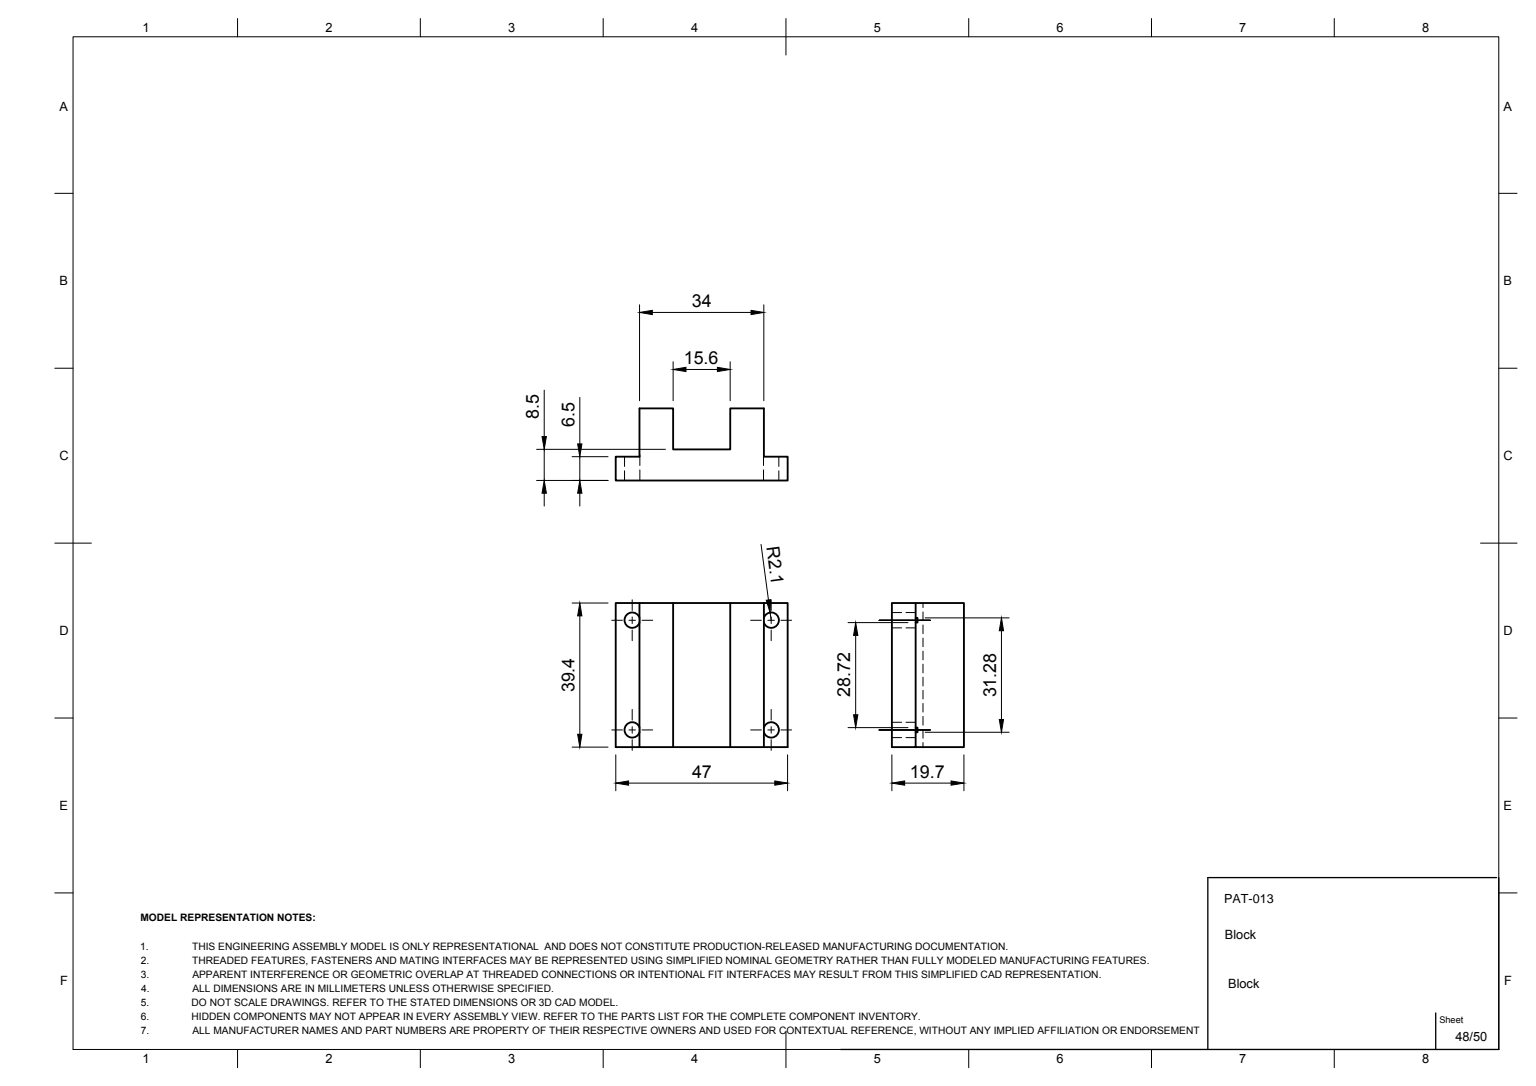
ISO-10303-21;
HEADER;
/* Generated by software containing ST-Developer
 * from STEP Tools, Inc. (www.steptools.com) 
 */

FILE_DESCRIPTION(
/* description */ ('Belt-driven linear axis on 2020 extrusion'),
/* implementation_level */ '2;1');

FILE_NAME(
/* name */ 'Block.step',
/* time_stamp */ '2026-10-28T03:26:09-07:00',
/* author */ (''),
/* organization */ (''),
/* preprocessor_version */ 'ST-DEVELOPER v20.2',
/* originating_system */ 'Autodesk Translation Framework v15.17.0.0',
/* authorisation */ '');

FILE_SCHEMA (('AUTOMOTIVE_DESIGN { 1 0 10303 214 3 1 1 }'));
ENDSEC;

DATA;
#10=MECHANICAL_DESIGN_GEOMETRIC_PRESENTATION_REPRESENTATION('',(#659),#20096);
#557=SHAPE_REPRESENTATION_RELATIONSHIP('SRR','None',#20358,#603);
#603=ADVANCED_BREP_SHAPE_REPRESENTATION('',(#714),#20089);
#659=STYLED_ITEM('',(#20629),#714);
#714=MANIFOLD_SOLID_BREP('Body1',#10973);
#880=FACE_BOUND('',#2573,.T.);
#881=FACE_BOUND('',#2574,.T.);
#882=FACE_BOUND('',#2575,.T.);
#883=FACE_BOUND('',#2576,.T.);
#1177=PLANE('',#12538);
#1178=PLANE('',#12544);
#1179=PLANE('',#12550);
#1180=PLANE('',#12556);
#1181=PLANE('',#12562);
#1182=PLANE('',#12563);
#1183=PLANE('',#12564);
#1184=PLANE('',#12565);
#1185=PLANE('',#12566);
#1186=PLANE('',#12567);
#1187=PLANE('',#12568);
#1188=PLANE('',#12569);
#1189=PLANE('',#12570);
#1190=PLANE('',#12571);
#1191=PLANE('',#12572);
#1192=PLANE('',#12573);
#1193=PLANE('',#12574);
#1194=PLANE('',#12575);
#1775=FACE_OUTER_BOUND('',#2559,.T.);
#1776=FACE_OUTER_BOUND('',#2560,.T.);
#1777=FACE_OUTER_BOUND('',#2561,.T.);
#1778=FACE_OUTER_BOUND('',#2562,.T.);
#1779=FACE_OUTER_BOUND('',#2563,.T.);
#1780=FACE_OUTER_BOUND('',#2564,.T.);
#1781=FACE_OUTER_BOUND('',#2565,.T.);
#1782=FACE_OUTER_BOUND('',#2566,.T.);
#1783=FACE_OUTER_BOUND('',#2567,.T.);
#1784=FACE_OUTER_BOUND('',#2568,.T.);
#1785=FACE_OUTER_BOUND('',#2569,.T.);
#1786=FACE_OUTER_BOUND('',#2570,.T.);
#1787=FACE_OUTER_BOUND('',#2571,.T.);
#1788=FACE_OUTER_BOUND('',#2572,.T.);
#1789=FACE_OUTER_BOUND('',#2577,.T.);
#1790=FACE_OUTER_BOUND('',#2578,.T.);
#1791=FACE_OUTER_BOUND('',#2579,.T.);
#1792=FACE_OUTER_BOUND('',#2580,.T.);
#1793=FACE_OUTER_BOUND('',#2581,.T.);
#1794=FACE_OUTER_BOUND('',#2582,.T.);
#1795=FACE_OUTER_BOUND('',#2583,.T.);
#1796=FACE_OUTER_BOUND('',#2584,.T.);
#2559=EDGE_LOOP('',(#9633,#9634));
#2560=EDGE_LOOP('',(#9635,#9636,#9637,#9638,#9639,#9640,#9641,#9642));
#2561=EDGE_LOOP('',(#9643,#9644));
#2562=EDGE_LOOP('',(#9645,#9646,#9647,#9648,#9649,#9650,#9651,#9652));
#2563=EDGE_LOOP('',(#9653,#9654));
#2564=EDGE_LOOP('',(#9655,#9656,#9657,#9658,#9659,#9660,#9661,#9662));
#2565=EDGE_LOOP('',(#9663,#9664));
#2566=EDGE_LOOP('',(#9665,#9666,#9667,#9668,#9669,#9670,#9671,#9672));
#2567=EDGE_LOOP('',(#9673,#9674,#9675,#9676,#9677,#9678,#9679,#9680,#9681,
#9682,#9683,#9684));
#2568=EDGE_LOOP('',(#9685,#9686,#9687,#9688,#9689,#9690,#9691,#9692,#9693,
#9694,#9695,#9696));
#2569=EDGE_LOOP('',(#9697,#9698,#9699,#9700,#9701,#9702,#9703,#9704,#9705,
#9706,#9707,#9708));
#2570=EDGE_LOOP('',(#9709,#9710,#9711,#9712,#9713,#9714,#9715,#9716,#9717,
#9718));
#2571=EDGE_LOOP('',(#9719,#9720,#9721,#9722));
#2572=EDGE_LOOP('',(#9723,#9724,#9725,#9726));
#2573=EDGE_LOOP('',(#9727));
#2574=EDGE_LOOP('',(#9728));
#2575=EDGE_LOOP('',(#9729));
#2576=EDGE_LOOP('',(#9730));
#2577=EDGE_LOOP('',(#9731,#9732,#9733,#9734));
#2578=EDGE_LOOP('',(#9735,#9736,#9737,#9738,#9739,#9740,#9741,#9742,#9743,
#9744));
#2579=EDGE_LOOP('',(#9745,#9746,#9747,#9748));
#2580=EDGE_LOOP('',(#9749,#9750,#9751,#9752));
#2581=EDGE_LOOP('',(#9753,#9754,#9755,#9756));
#2582=EDGE_LOOP('',(#9757,#9758,#9759,#9760));
#2583=EDGE_LOOP('',(#9761,#9762,#9763,#9764));
#2584=EDGE_LOOP('',(#9765,#9766,#9767,#9768,#9769,#9770,#9771,#9772,#9773,
#9774,#9775,#9776));
#3344=LINE('',#19423,#4201);
#3345=LINE('',#19427,#4202);
#3346=LINE('',#19431,#4203);
#3347=LINE('',#19435,#4204);
#3348=LINE('',#19439,#4205);
#3349=LINE('',#19443,#4206);
#3350=LINE('',#19447,#4207);
#3351=LINE('',#19451,#4208);
#3352=LINE('',#19455,#4209);
#3353=LINE('',#19459,#4210);
#3354=LINE('',#19463,#4211);
#3355=LINE('',#19467,#4212);
#3356=LINE('',#19471,#4213);
#3357=LINE('',#19475,#4214);
#3358=LINE('',#19479,#4215);
#3359=LINE('',#19483,#4216);
#3360=LINE('',#19485,#4217);
#3361=LINE('',#19487,#4218);
#3362=LINE('',#19489,#4219);
#3363=LINE('',#19491,#4220);
#3364=LINE('',#19493,#4221);
#3365=LINE('',#19494,#4222);
#3366=LINE('',#19496,#4223);
#3367=LINE('',#19498,#4224);
#3368=LINE('',#19500,#4225);
#3369=LINE('',#19502,#4226);
#3370=LINE('',#19504,#4227);
#3371=LINE('',#19505,#4228);
#3372=LINE('',#19508,#4229);
#3373=LINE('',#19510,#4230);
#3374=LINE('',#19512,#4231);
#3375=LINE('',#19514,#4232);
#3376=LINE('',#19515,#4233);
#3377=LINE('',#19517,#4234);
#3378=LINE('',#19519,#4235);
#3379=LINE('',#19521,#4236);
#3380=LINE('',#19523,#4237);
#3381=LINE('',#19524,#4238);
#3382=LINE('',#19527,#4239);
#3383=LINE('',#19528,#4240);
#3384=LINE('',#19531,#4241);
#3385=LINE('',#19532,#4242);
#3386=LINE('',#19535,#4243);
#3387=LINE('',#19536,#4244);
#3388=LINE('',#19539,#4245);
#3389=LINE('',#19540,#4246);
#3390=LINE('',#19542,#4247);
#3391=LINE('',#19545,#4248);
#3392=LINE('',#19546,#4249);
#3393=LINE('',#19549,#4250);
#3394=LINE('',#19550,#4251);
#3395=LINE('',#19553,#4252);
#3396=LINE('',#19554,#4253);
#3397=LINE('',#19557,#4254);
#3398=LINE('',#19558,#4255);
#3399=LINE('',#19560,#4256);
#4201=VECTOR('',#15562,1.);
#4202=VECTOR('',#15567,1.);
#4203=VECTOR('',#15570,0.21);
#4204=VECTOR('',#15575,1.);
#4205=VECTOR('',#15578,1.);
#4206=VECTOR('',#15583,1.);
#4207=VECTOR('',#15586,0.21);
#4208=VECTOR('',#15591,1.);
#4209=VECTOR('',#15594,1.);
#4210=VECTOR('',#15599,1.);
#4211=VECTOR('',#15602,0.21);
#4212=VECTOR('',#15607,1.);
#4213=VECTOR('',#15610,1.);
#4214=VECTOR('',#15615,1.);
#4215=VECTOR('',#15618,0.21);
#4216=VECTOR('',#15623,1.);
#4217=VECTOR('',#15626,1.);
#4218=VECTOR('',#15627,1.);
#4219=VECTOR('',#15628,1.);
#4220=VECTOR('',#15629,1.);
#4221=VECTOR('',#15630,1.);
#4222=VECTOR('',#15631,1.);
#4223=VECTOR('',#15634,1.);
#4224=VECTOR('',#15635,1.);
#4225=VECTOR('',#15636,1.);
#4226=VECTOR('',#15637,1.);
#4227=VECTOR('',#15638,1.);
#4228=VECTOR('',#15639,1.);
#4229=VECTOR('',#15642,1.);
#4230=VECTOR('',#15643,1.);
#4231=VECTOR('',#15644,1.);
#4232=VECTOR('',#15645,1.);
#4233=VECTOR('',#15646,1.);
#4234=VECTOR('',#15647,1.);
#4235=VECTOR('',#15648,1.);
#4236=VECTOR('',#15649,1.);
#4237=VECTOR('',#15650,1.);
#4238=VECTOR('',#15651,1.);
#4239=VECTOR('',#15654,1.);
#4240=VECTOR('',#15655,1.);
#4241=VECTOR('',#15658,1.);
#4242=VECTOR('',#15659,1.);
#4243=VECTOR('',#15662,1.);
#4244=VECTOR('',#15663,1.);
#4245=VECTOR('',#15666,1.);
#4246=VECTOR('',#15667,1.);
#4247=VECTOR('',#15670,1.);
#4248=VECTOR('',#15673,1.);
#4249=VECTOR('',#15674,1.);
#4250=VECTOR('',#15677,1.);
#4251=VECTOR('',#15678,1.);
#4252=VECTOR('',#15681,1.);
#4253=VECTOR('',#15682,1.);
#4254=VECTOR('',#15685,1.);
#4255=VECTOR('',#15686,1.);
#4256=VECTOR('',#15689,1.);
#4848=CIRCLE('',#12539,0.21);
#4849=CIRCLE('',#12541,0.21);
#4850=CIRCLE('',#12542,0.21);
#4851=CIRCLE('',#12543,0.21);
#4852=CIRCLE('',#12545,0.21);
#4853=CIRCLE('',#12547,0.21);
#4854=CIRCLE('',#12548,0.21);
#4855=CIRCLE('',#12549,0.21);
#4856=CIRCLE('',#12551,0.21);
#4857=CIRCLE('',#12553,0.21);
#4858=CIRCLE('',#12554,0.21);
#4859=CIRCLE('',#12555,0.21);
#4860=CIRCLE('',#12557,0.21);
#4861=CIRCLE('',#12559,0.21);
#4862=CIRCLE('',#12560,0.21);
#4863=CIRCLE('',#12561,0.21);
#5697=VERTEX_POINT('',#19421);
#5698=VERTEX_POINT('',#19422);
#5699=VERTEX_POINT('',#19426);
#5700=VERTEX_POINT('',#19428);
#5701=VERTEX_POINT('',#19430);
#5702=VERTEX_POINT('',#19433);
#5703=VERTEX_POINT('',#19437);
#5704=VERTEX_POINT('',#19438);
#5705=VERTEX_POINT('',#19442);
#5706=VERTEX_POINT('',#19444);
#5707=VERTEX_POINT('',#19446);
#5708=VERTEX_POINT('',#19449);
#5709=VERTEX_POINT('',#19453);
#5710=VERTEX_POINT('',#19454);
#5711=VERTEX_POINT('',#19458);
#5712=VERTEX_POINT('',#19460);
#5713=VERTEX_POINT('',#19462);
#5714=VERTEX_POINT('',#19465);
#5715=VERTEX_POINT('',#19469);
#5716=VERTEX_POINT('',#19470);
#5717=VERTEX_POINT('',#19474);
#5718=VERTEX_POINT('',#19476);
#5719=VERTEX_POINT('',#19478);
#5720=VERTEX_POINT('',#19481);
#5721=VERTEX_POINT('',#19486);
#5722=VERTEX_POINT('',#19488);
#5723=VERTEX_POINT('',#19490);
#5724=VERTEX_POINT('',#19492);
#5725=VERTEX_POINT('',#19497);
#5726=VERTEX_POINT('',#19499);
#5727=VERTEX_POINT('',#19501);
#5728=VERTEX_POINT('',#19503);
#5729=VERTEX_POINT('',#19507);
#5730=VERTEX_POINT('',#19509);
#5731=VERTEX_POINT('',#19511);
#5732=VERTEX_POINT('',#19513);
#5733=VERTEX_POINT('',#19516);
#5734=VERTEX_POINT('',#19518);
#5735=VERTEX_POINT('',#19520);
#5736=VERTEX_POINT('',#19522);
#5737=VERTEX_POINT('',#19526);
#5738=VERTEX_POINT('',#19530);
#5739=VERTEX_POINT('',#19534);
#5740=VERTEX_POINT('',#19538);
#5741=VERTEX_POINT('',#19544);
#5742=VERTEX_POINT('',#19548);
#5743=VERTEX_POINT('',#19552);
#5744=VERTEX_POINT('',#19556);
#7031=EDGE_CURVE('',#5697,#5698,#3344,.T.);
#7032=EDGE_CURVE('',#5697,#5698,#4848,.T.);
#7033=EDGE_CURVE('',#5699,#5697,#3345,.T.);
#7034=EDGE_CURVE('',#5700,#5699,#4849,.T.);
#7035=EDGE_CURVE('',#5700,#5701,#3346,.T.);
#7036=EDGE_CURVE('',#5701,#5701,#4850,.T.);
#7037=EDGE_CURVE('',#5702,#5700,#4851,.T.);
#7038=EDGE_CURVE('',#5698,#5702,#3347,.T.);
#7039=EDGE_CURVE('',#5703,#5704,#3348,.T.);
#7040=EDGE_CURVE('',#5703,#5704,#4852,.T.);
#7041=EDGE_CURVE('',#5705,#5703,#3349,.T.);
#7042=EDGE_CURVE('',#5706,#5705,#4853,.T.);
#7043=EDGE_CURVE('',#5706,#5707,#3350,.T.);
#7044=EDGE_CURVE('',#5707,#5707,#4854,.T.);
#7045=EDGE_CURVE('',#5708,#5706,#4855,.T.);
#7046=EDGE_CURVE('',#5704,#5708,#3351,.T.);
#7047=EDGE_CURVE('',#5709,#5710,#3352,.T.);
#7048=EDGE_CURVE('',#5709,#5710,#4856,.T.);
#7049=EDGE_CURVE('',#5711,#5709,#3353,.T.);
#7050=EDGE_CURVE('',#5712,#5711,#4857,.T.);
#7051=EDGE_CURVE('',#5712,#5713,#3354,.T.);
#7052=EDGE_CURVE('',#5713,#5713,#4858,.T.);
#7053=EDGE_CURVE('',#5714,#5712,#4859,.T.);
#7054=EDGE_CURVE('',#5710,#5714,#3355,.T.);
#7055=EDGE_CURVE('',#5715,#5716,#3356,.T.);
#7056=EDGE_CURVE('',#5715,#5716,#4860,.T.);
#7057=EDGE_CURVE('',#5717,#5715,#3357,.T.);
#7058=EDGE_CURVE('',#5718,#5717,#4861,.T.);
#7059=EDGE_CURVE('',#5718,#5719,#3358,.T.);
#7060=EDGE_CURVE('',#5719,#5719,#4862,.T.);
#7061=EDGE_CURVE('',#5720,#5718,#4863,.T.);
#7062=EDGE_CURVE('',#5716,#5720,#3359,.T.);
#7063=EDGE_CURVE('',#5702,#5711,#3360,.T.);
#7064=EDGE_CURVE('',#5714,#5721,#3361,.T.);
#7065=EDGE_CURVE('',#5722,#5721,#3362,.T.);
#7066=EDGE_CURVE('',#5722,#5723,#3363,.T.);
#7067=EDGE_CURVE('',#5724,#5723,#3364,.T.);
#7068=EDGE_CURVE('',#5724,#5699,#3365,.T.);
#7069=EDGE_CURVE('',#5708,#5717,#3366,.T.);
#7070=EDGE_CURVE('',#5720,#5725,#3367,.T.);
#7071=EDGE_CURVE('',#5726,#5725,#3368,.T.);
#7072=EDGE_CURVE('',#5727,#5726,#3369,.T.);
#7073=EDGE_CURVE('',#5728,#5727,#3370,.T.);
#7074=EDGE_CURVE('',#5728,#5705,#3371,.T.);
#7075=EDGE_CURVE('',#5721,#5729,#3372,.T.);
#7076=EDGE_CURVE('',#5729,#5730,#3373,.T.);
#7077=EDGE_CURVE('',#5730,#5731,#3374,.T.);
#7078=EDGE_CURVE('',#5731,#5732,#3375,.T.);
#7079=EDGE_CURVE('',#5732,#5728,#3376,.T.);
#7080=EDGE_CURVE('',#5727,#5733,#3377,.T.);
#7081=EDGE_CURVE('',#5733,#5734,#3378,.T.);
#7082=EDGE_CURVE('',#5734,#5735,#3379,.T.);
#7083=EDGE_CURVE('',#5735,#5736,#3380,.T.);
#7084=EDGE_CURVE('',#5736,#5722,#3381,.T.);
#7085=EDGE_CURVE('',#5737,#5724,#3382,.T.);
#7086=EDGE_CURVE('',#5729,#5737,#3383,.T.);
#7087=EDGE_CURVE('',#5738,#5737,#3384,.T.);
#7088=EDGE_CURVE('',#5730,#5738,#3385,.T.);
#7089=EDGE_CURVE('',#5739,#5738,#3386,.T.);
#7090=EDGE_CURVE('',#5731,#5739,#3387,.T.);
#7091=EDGE_CURVE('',#5740,#5739,#3388,.T.);
#7092=EDGE_CURVE('',#5732,#5740,#3389,.T.);
#7093=EDGE_CURVE('',#5725,#5740,#3390,.T.);
#7094=EDGE_CURVE('',#5741,#5726,#3391,.T.);
#7095=EDGE_CURVE('',#5733,#5741,#3392,.T.);
#7096=EDGE_CURVE('',#5742,#5741,#3393,.T.);
#7097=EDGE_CURVE('',#5734,#5742,#3394,.T.);
#7098=EDGE_CURVE('',#5743,#5742,#3395,.T.);
#7099=EDGE_CURVE('',#5735,#5743,#3396,.T.);
#7100=EDGE_CURVE('',#5744,#5743,#3397,.T.);
#7101=EDGE_CURVE('',#5736,#5744,#3398,.T.);
#7102=EDGE_CURVE('',#5723,#5744,#3399,.T.);
#9633=ORIENTED_EDGE('',*,*,#7031,.F.);
#9634=ORIENTED_EDGE('',*,*,#7032,.T.);
#9635=ORIENTED_EDGE('',*,*,#7033,.F.);
#9636=ORIENTED_EDGE('',*,*,#7034,.F.);
#9637=ORIENTED_EDGE('',*,*,#7035,.T.);
#9638=ORIENTED_EDGE('',*,*,#7036,.F.);
#9639=ORIENTED_EDGE('',*,*,#7035,.F.);
#9640=ORIENTED_EDGE('',*,*,#7037,.F.);
#9641=ORIENTED_EDGE('',*,*,#7038,.F.);
#9642=ORIENTED_EDGE('',*,*,#7032,.F.);
#9643=ORIENTED_EDGE('',*,*,#7039,.F.);
#9644=ORIENTED_EDGE('',*,*,#7040,.T.);
#9645=ORIENTED_EDGE('',*,*,#7041,.F.);
#9646=ORIENTED_EDGE('',*,*,#7042,.F.);
#9647=ORIENTED_EDGE('',*,*,#7043,.T.);
#9648=ORIENTED_EDGE('',*,*,#7044,.F.);
#9649=ORIENTED_EDGE('',*,*,#7043,.F.);
#9650=ORIENTED_EDGE('',*,*,#7045,.F.);
#9651=ORIENTED_EDGE('',*,*,#7046,.F.);
#9652=ORIENTED_EDGE('',*,*,#7040,.F.);
#9653=ORIENTED_EDGE('',*,*,#7047,.F.);
#9654=ORIENTED_EDGE('',*,*,#7048,.T.);
#9655=ORIENTED_EDGE('',*,*,#7049,.F.);
#9656=ORIENTED_EDGE('',*,*,#7050,.F.);
#9657=ORIENTED_EDGE('',*,*,#7051,.T.);
#9658=ORIENTED_EDGE('',*,*,#7052,.F.);
#9659=ORIENTED_EDGE('',*,*,#7051,.F.);
#9660=ORIENTED_EDGE('',*,*,#7053,.F.);
#9661=ORIENTED_EDGE('',*,*,#7054,.F.);
#9662=ORIENTED_EDGE('',*,*,#7048,.F.);
#9663=ORIENTED_EDGE('',*,*,#7055,.F.);
#9664=ORIENTED_EDGE('',*,*,#7056,.T.);
#9665=ORIENTED_EDGE('',*,*,#7057,.F.);
#9666=ORIENTED_EDGE('',*,*,#7058,.F.);
#9667=ORIENTED_EDGE('',*,*,#7059,.T.);
#9668=ORIENTED_EDGE('',*,*,#7060,.F.);
#9669=ORIENTED_EDGE('',*,*,#7059,.F.);
#9670=ORIENTED_EDGE('',*,*,#7061,.F.);
#9671=ORIENTED_EDGE('',*,*,#7062,.F.);
#9672=ORIENTED_EDGE('',*,*,#7056,.F.);
#9673=ORIENTED_EDGE('',*,*,#7033,.T.);
#9674=ORIENTED_EDGE('',*,*,#7031,.T.);
#9675=ORIENTED_EDGE('',*,*,#7038,.T.);
#9676=ORIENTED_EDGE('',*,*,#7063,.T.);
#9677=ORIENTED_EDGE('',*,*,#7049,.T.);
#9678=ORIENTED_EDGE('',*,*,#7047,.T.);
#9679=ORIENTED_EDGE('',*,*,#7054,.T.);
#9680=ORIENTED_EDGE('',*,*,#7064,.T.);
#9681=ORIENTED_EDGE('',*,*,#7065,.F.);
#9682=ORIENTED_EDGE('',*,*,#7066,.T.);
#9683=ORIENTED_EDGE('',*,*,#7067,.F.);
#9684=ORIENTED_EDGE('',*,*,#7068,.T.);
#9685=ORIENTED_EDGE('',*,*,#7041,.T.);
#9686=ORIENTED_EDGE('',*,*,#7039,.T.);
#9687=ORIENTED_EDGE('',*,*,#7046,.T.);
#9688=ORIENTED_EDGE('',*,*,#7069,.T.);
#9689=ORIENTED_EDGE('',*,*,#7057,.T.);
#9690=ORIENTED_EDGE('',*,*,#7055,.T.);
#9691=ORIENTED_EDGE('',*,*,#7062,.T.);
#9692=ORIENTED_EDGE('',*,*,#7070,.T.);
#9693=ORIENTED_EDGE('',*,*,#7071,.F.);
#9694=ORIENTED_EDGE('',*,*,#7072,.F.);
#9695=ORIENTED_EDGE('',*,*,#7073,.F.);
#9696=ORIENTED_EDGE('',*,*,#7074,.T.);
#9697=ORIENTED_EDGE('',*,*,#7065,.T.);
#9698=ORIENTED_EDGE('',*,*,#7075,.T.);
#9699=ORIENTED_EDGE('',*,*,#7076,.T.);
#9700=ORIENTED_EDGE('',*,*,#7077,.T.);
#9701=ORIENTED_EDGE('',*,*,#7078,.T.);
#9702=ORIENTED_EDGE('',*,*,#7079,.T.);
#9703=ORIENTED_EDGE('',*,*,#7073,.T.);
#9704=ORIENTED_EDGE('',*,*,#7080,.T.);
#9705=ORIENTED_EDGE('',*,*,#7081,.T.);
#9706=ORIENTED_EDGE('',*,*,#7082,.T.);
#9707=ORIENTED_EDGE('',*,*,#7083,.T.);
#9708=ORIENTED_EDGE('',*,*,#7084,.T.);
#9709=ORIENTED_EDGE('',*,*,#7037,.T.);
#9710=ORIENTED_EDGE('',*,*,#7034,.T.);
#9711=ORIENTED_EDGE('',*,*,#7068,.F.);
#9712=ORIENTED_EDGE('',*,*,#7085,.F.);
#9713=ORIENTED_EDGE('',*,*,#7086,.F.);
#9714=ORIENTED_EDGE('',*,*,#7075,.F.);
#9715=ORIENTED_EDGE('',*,*,#7064,.F.);
#9716=ORIENTED_EDGE('',*,*,#7053,.T.);
#9717=ORIENTED_EDGE('',*,*,#7050,.T.);
#9718=ORIENTED_EDGE('',*,*,#7063,.F.);
#9719=ORIENTED_EDGE('',*,*,#7086,.T.);
#9720=ORIENTED_EDGE('',*,*,#7087,.F.);
#9721=ORIENTED_EDGE('',*,*,#7088,.F.);
#9722=ORIENTED_EDGE('',*,*,#7076,.F.);
#9723=ORIENTED_EDGE('',*,*,#7088,.T.);
#9724=ORIENTED_EDGE('',*,*,#7089,.F.);
#9725=ORIENTED_EDGE('',*,*,#7090,.F.);
#9726=ORIENTED_EDGE('',*,*,#7077,.F.);
#9727=ORIENTED_EDGE('',*,*,#7036,.T.);
#9728=ORIENTED_EDGE('',*,*,#7044,.T.);
#9729=ORIENTED_EDGE('',*,*,#7052,.T.);
#9730=ORIENTED_EDGE('',*,*,#7060,.T.);
#9731=ORIENTED_EDGE('',*,*,#7090,.T.);
#9732=ORIENTED_EDGE('',*,*,#7091,.F.);
#9733=ORIENTED_EDGE('',*,*,#7092,.F.);
#9734=ORIENTED_EDGE('',*,*,#7078,.F.);
#9735=ORIENTED_EDGE('',*,*,#7045,.T.);
#9736=ORIENTED_EDGE('',*,*,#7042,.T.);
#9737=ORIENTED_EDGE('',*,*,#7074,.F.);
#9738=ORIENTED_EDGE('',*,*,#7079,.F.);
#9739=ORIENTED_EDGE('',*,*,#7092,.T.);
#9740=ORIENTED_EDGE('',*,*,#7093,.F.);
#9741=ORIENTED_EDGE('',*,*,#7070,.F.);
#9742=ORIENTED_EDGE('',*,*,#7061,.T.);
#9743=ORIENTED_EDGE('',*,*,#7058,.T.);
#9744=ORIENTED_EDGE('',*,*,#7069,.F.);
#9745=ORIENTED_EDGE('',*,*,#7072,.T.);
#9746=ORIENTED_EDGE('',*,*,#7094,.F.);
#9747=ORIENTED_EDGE('',*,*,#7095,.F.);
#9748=ORIENTED_EDGE('',*,*,#7080,.F.);
#9749=ORIENTED_EDGE('',*,*,#7095,.T.);
#9750=ORIENTED_EDGE('',*,*,#7096,.F.);
#9751=ORIENTED_EDGE('',*,*,#7097,.F.);
#9752=ORIENTED_EDGE('',*,*,#7081,.F.);
#9753=ORIENTED_EDGE('',*,*,#7097,.T.);
#9754=ORIENTED_EDGE('',*,*,#7098,.F.);
#9755=ORIENTED_EDGE('',*,*,#7099,.F.);
#9756=ORIENTED_EDGE('',*,*,#7082,.F.);
#9757=ORIENTED_EDGE('',*,*,#7099,.T.);
#9758=ORIENTED_EDGE('',*,*,#7100,.F.);
#9759=ORIENTED_EDGE('',*,*,#7101,.F.);
#9760=ORIENTED_EDGE('',*,*,#7083,.F.);
#9761=ORIENTED_EDGE('',*,*,#7101,.T.);
#9762=ORIENTED_EDGE('',*,*,#7102,.F.);
#9763=ORIENTED_EDGE('',*,*,#7066,.F.);
#9764=ORIENTED_EDGE('',*,*,#7084,.F.);
#9765=ORIENTED_EDGE('',*,*,#7067,.T.);
#9766=ORIENTED_EDGE('',*,*,#7102,.T.);
#9767=ORIENTED_EDGE('',*,*,#7100,.T.);
#9768=ORIENTED_EDGE('',*,*,#7098,.T.);
#9769=ORIENTED_EDGE('',*,*,#7096,.T.);
#9770=ORIENTED_EDGE('',*,*,#7094,.T.);
#9771=ORIENTED_EDGE('',*,*,#7071,.T.);
#9772=ORIENTED_EDGE('',*,*,#7093,.T.);
#9773=ORIENTED_EDGE('',*,*,#7091,.T.);
#9774=ORIENTED_EDGE('',*,*,#7089,.T.);
#9775=ORIENTED_EDGE('',*,*,#7087,.T.);
#9776=ORIENTED_EDGE('',*,*,#7085,.T.);
#10289=CYLINDRICAL_SURFACE('',#12540,0.21);
#10290=CYLINDRICAL_SURFACE('',#12546,0.21);
#10291=CYLINDRICAL_SURFACE('',#12552,0.21);
#10292=CYLINDRICAL_SURFACE('',#12558,0.21);
#10826=ADVANCED_FACE('',(#1775),#1177,.T.);
#10827=ADVANCED_FACE('',(#1776),#10289,.F.);
#10828=ADVANCED_FACE('',(#1777),#1178,.T.);
#10829=ADVANCED_FACE('',(#1778),#10290,.F.);
#10830=ADVANCED_FACE('',(#1779),#1179,.T.);
#10831=ADVANCED_FACE('',(#1780),#10291,.F.);
#10832=ADVANCED_FACE('',(#1781),#1180,.T.);
#10833=ADVANCED_FACE('',(#1782),#10292,.F.);
#10834=ADVANCED_FACE('',(#1783),#1181,.T.);
#10835=ADVANCED_FACE('',(#1784),#1182,.T.);
#10836=ADVANCED_FACE('',(#1785),#1183,.T.);
#10837=ADVANCED_FACE('',(#1786),#1184,.T.);
#10838=ADVANCED_FACE('',(#1787),#1185,.T.);
#10839=ADVANCED_FACE('',(#1788,#880,#881,#882,#883),#1186,.T.);
#10840=ADVANCED_FACE('',(#1789),#1187,.T.);
#10841=ADVANCED_FACE('',(#1790),#1188,.T.);
#10842=ADVANCED_FACE('',(#1791),#1189,.T.);
#10843=ADVANCED_FACE('',(#1792),#1190,.T.);
#10844=ADVANCED_FACE('',(#1793),#1191,.T.);
#10845=ADVANCED_FACE('',(#1794),#1192,.T.);
#10846=ADVANCED_FACE('',(#1795),#1193,.T.);
#10847=ADVANCED_FACE('',(#1796),#1194,.T.);
#10973=CLOSED_SHELL('',(#10826,#10827,#10828,#10829,#10830,#10831,#10832,
#10833,#10834,#10835,#10836,#10837,#10838,#10839,#10840,#10841,#10842,#10843,
#10844,#10845,#10846,#10847));
#12537=AXIS2_PLACEMENT_3D('',#19419,#15558,#15559);
#12538=AXIS2_PLACEMENT_3D('',#19420,#15560,#15561);
#12539=AXIS2_PLACEMENT_3D('',#19424,#15563,#15564);
#12540=AXIS2_PLACEMENT_3D('',#19425,#15565,#15566);
#12541=AXIS2_PLACEMENT_3D('',#19429,#15568,#15569);
#12542=AXIS2_PLACEMENT_3D('',#19432,#15571,#15572);
#12543=AXIS2_PLACEMENT_3D('',#19434,#15573,#15574);
#12544=AXIS2_PLACEMENT_3D('',#19436,#15576,#15577);
#12545=AXIS2_PLACEMENT_3D('',#19440,#15579,#15580);
#12546=AXIS2_PLACEMENT_3D('',#19441,#15581,#15582);
#12547=AXIS2_PLACEMENT_3D('',#19445,#15584,#15585);
#12548=AXIS2_PLACEMENT_3D('',#19448,#15587,#15588);
#12549=AXIS2_PLACEMENT_3D('',#19450,#15589,#15590);
#12550=AXIS2_PLACEMENT_3D('',#19452,#15592,#15593);
#12551=AXIS2_PLACEMENT_3D('',#19456,#15595,#15596);
#12552=AXIS2_PLACEMENT_3D('',#19457,#15597,#15598);
#12553=AXIS2_PLACEMENT_3D('',#19461,#15600,#15601);
#12554=AXIS2_PLACEMENT_3D('',#19464,#15603,#15604);
#12555=AXIS2_PLACEMENT_3D('',#19466,#15605,#15606);
#12556=AXIS2_PLACEMENT_3D('',#19468,#15608,#15609);
#12557=AXIS2_PLACEMENT_3D('',#19472,#15611,#15612);
#12558=AXIS2_PLACEMENT_3D('',#19473,#15613,#15614);
#12559=AXIS2_PLACEMENT_3D('',#19477,#15616,#15617);
#12560=AXIS2_PLACEMENT_3D('',#19480,#15619,#15620);
#12561=AXIS2_PLACEMENT_3D('',#19482,#15621,#15622);
#12562=AXIS2_PLACEMENT_3D('',#19484,#15624,#15625);
#12563=AXIS2_PLACEMENT_3D('',#19495,#15632,#15633);
#12564=AXIS2_PLACEMENT_3D('',#19506,#15640,#15641);
#12565=AXIS2_PLACEMENT_3D('',#19525,#15652,#15653);
#12566=AXIS2_PLACEMENT_3D('',#19529,#15656,#15657);
#12567=AXIS2_PLACEMENT_3D('',#19533,#15660,#15661);
#12568=AXIS2_PLACEMENT_3D('',#19537,#15664,#15665);
#12569=AXIS2_PLACEMENT_3D('',#19541,#15668,#15669);
#12570=AXIS2_PLACEMENT_3D('',#19543,#15671,#15672);
#12571=AXIS2_PLACEMENT_3D('',#19547,#15675,#15676);
#12572=AXIS2_PLACEMENT_3D('',#19551,#15679,#15680);
#12573=AXIS2_PLACEMENT_3D('',#19555,#15683,#15684);
#12574=AXIS2_PLACEMENT_3D('',#19559,#15687,#15688);
#12575=AXIS2_PLACEMENT_3D('',#19561,#15690,#15691);
#15558=DIRECTION('axis',(0.,0.,1.));
#15559=DIRECTION('refdir',(1.,0.,0.));
#15560=DIRECTION('center_axis',(0.,0.,1.));
#15561=DIRECTION('ref_axis',(1.,0.,0.));
#15562=DIRECTION('',(-1.,0.,0.));
#15563=DIRECTION('center_axis',(0.,0.,1.));
#15564=DIRECTION('ref_axis',(1.,0.,0.));
#15565=DIRECTION('center_axis',(0.,0.,1.));
#15566=DIRECTION('ref_axis',(1.,0.,0.));
#15567=DIRECTION('',(0.,0.,-1.));
#15568=DIRECTION('center_axis',(0.,0.,1.));
#15569=DIRECTION('ref_axis',(1.,0.,0.));
#15570=DIRECTION('',(0.,0.,1.));
#15571=DIRECTION('center_axis',(0.,0.,-1.));
#15572=DIRECTION('ref_axis',(1.,0.,0.));
#15573=DIRECTION('center_axis',(0.,0.,1.));
#15574=DIRECTION('ref_axis',(1.,0.,0.));
#15575=DIRECTION('',(0.,0.,1.));
#15576=DIRECTION('center_axis',(0.,0.,1.));
#15577=DIRECTION('ref_axis',(1.,0.,0.));
#15578=DIRECTION('',(1.,0.,0.));
#15579=DIRECTION('center_axis',(0.,0.,1.));
#15580=DIRECTION('ref_axis',(1.,0.,0.));
#15581=DIRECTION('center_axis',(0.,0.,1.));
#15582=DIRECTION('ref_axis',(1.,0.,0.));
#15583=DIRECTION('',(0.,0.,-1.));
#15584=DIRECTION('center_axis',(0.,0.,1.));
#15585=DIRECTION('ref_axis',(1.,0.,0.));
#15586=DIRECTION('',(0.,0.,1.));
#15587=DIRECTION('center_axis',(0.,0.,-1.));
#15588=DIRECTION('ref_axis',(1.,0.,0.));
#15589=DIRECTION('center_axis',(0.,0.,1.));
#15590=DIRECTION('ref_axis',(1.,0.,0.));
#15591=DIRECTION('',(0.,0.,1.));
#15592=DIRECTION('center_axis',(0.,0.,1.));
#15593=DIRECTION('ref_axis',(1.,0.,0.));
#15594=DIRECTION('',(-1.,0.,0.));
#15595=DIRECTION('center_axis',(0.,0.,1.));
#15596=DIRECTION('ref_axis',(1.,0.,0.));
#15597=DIRECTION('center_axis',(0.,0.,1.));
#15598=DIRECTION('ref_axis',(1.,0.,0.));
#15599=DIRECTION('',(0.,0.,-1.));
#15600=DIRECTION('center_axis',(0.,0.,1.));
#15601=DIRECTION('ref_axis',(1.,0.,0.));
#15602=DIRECTION('',(0.,0.,1.));
#15603=DIRECTION('center_axis',(0.,0.,-1.));
#15604=DIRECTION('ref_axis',(1.,0.,0.));
#15605=DIRECTION('center_axis',(0.,0.,1.));
#15606=DIRECTION('ref_axis',(1.,0.,0.));
#15607=DIRECTION('',(0.,0.,1.));
#15608=DIRECTION('center_axis',(0.,0.,1.));
#15609=DIRECTION('ref_axis',(1.,0.,0.));
#15610=DIRECTION('',(1.,0.,0.));
#15611=DIRECTION('center_axis',(0.,0.,1.));
#15612=DIRECTION('ref_axis',(1.,0.,0.));
#15613=DIRECTION('center_axis',(0.,0.,1.));
#15614=DIRECTION('ref_axis',(1.,0.,0.));
#15615=DIRECTION('',(0.,0.,-1.));
#15616=DIRECTION('center_axis',(0.,0.,1.));
#15617=DIRECTION('ref_axis',(1.,0.,0.));
#15618=DIRECTION('',(0.,0.,1.));
#15619=DIRECTION('center_axis',(0.,0.,-1.));
#15620=DIRECTION('ref_axis',(1.,0.,0.));
#15621=DIRECTION('center_axis',(0.,0.,1.));
#15622=DIRECTION('ref_axis',(1.,0.,0.));
#15623=DIRECTION('',(0.,0.,1.));
#15624=DIRECTION('center_axis',(0.,-1.,0.));
#15625=DIRECTION('ref_axis',(0.,0.,-1.));
#15626=DIRECTION('',(-1.,0.,0.));
#15627=DIRECTION('',(-1.,0.,0.));
#15628=DIRECTION('',(0.,0.,1.));
#15629=DIRECTION('',(1.,0.,0.));
#15630=DIRECTION('',(0.,0.,-1.));
#15631=DIRECTION('',(-1.,0.,0.));
#15632=DIRECTION('center_axis',(0.,1.,0.));
#15633=DIRECTION('ref_axis',(0.,0.,1.));
#15634=DIRECTION('',(1.,0.,0.));
#15635=DIRECTION('',(1.,0.,0.));
#15636=DIRECTION('',(0.,0.,1.));
#15637=DIRECTION('',(1.,0.,0.));
#15638=DIRECTION('',(0.,0.,-1.));
#15639=DIRECTION('',(1.,0.,0.));
#15640=DIRECTION('center_axis',(-1.,0.,0.));
#15641=DIRECTION('ref_axis',(0.,0.,1.));
#15642=DIRECTION('',(0.,-1.,0.));
#15643=DIRECTION('',(0.,0.,1.));
#15644=DIRECTION('',(0.,1.,0.));
#15645=DIRECTION('',(0.,0.,-1.));
#15646=DIRECTION('',(0.,-1.,0.));
#15647=DIRECTION('',(0.,-1.,0.));
#15648=DIRECTION('',(0.,0.,1.));
#15649=DIRECTION('',(0.,-1.,0.));
#15650=DIRECTION('',(0.,0.,-1.));
#15651=DIRECTION('',(0.,-1.,0.));
#15652=DIRECTION('center_axis',(0.,0.,-1.));
#15653=DIRECTION('ref_axis',(0.,1.,0.));
#15654=DIRECTION('',(0.,1.,0.));
#15655=DIRECTION('',(1.,0.,0.));
#15656=DIRECTION('center_axis',(0.,-1.,0.));
#15657=DIRECTION('ref_axis',(0.,0.,-1.));
#15658=DIRECTION('',(0.,0.,-1.));
#15659=DIRECTION('',(1.,0.,0.));
#15660=DIRECTION('center_axis',(0.,0.,1.));
#15661=DIRECTION('ref_axis',(0.,-1.,0.));
#15662=DIRECTION('',(0.,-1.,0.));
#15663=DIRECTION('',(1.,0.,0.));
#15664=DIRECTION('center_axis',(0.,1.,0.));
#15665=DIRECTION('ref_axis',(0.,0.,1.));
#15666=DIRECTION('',(0.,0.,1.));
#15667=DIRECTION('',(1.,0.,0.));
#15668=DIRECTION('center_axis',(0.,0.,-1.));
#15669=DIRECTION('ref_axis',(0.,1.,0.));
#15670=DIRECTION('',(0.,1.,0.));
#15671=DIRECTION('center_axis',(0.,0.,-1.));
#15672=DIRECTION('ref_axis',(0.,1.,0.));
#15673=DIRECTION('',(0.,1.,0.));
#15674=DIRECTION('',(1.,0.,0.));
#15675=DIRECTION('center_axis',(0.,-1.,0.));
#15676=DIRECTION('ref_axis',(0.,0.,-1.));
#15677=DIRECTION('',(0.,0.,-1.));
#15678=DIRECTION('',(1.,0.,0.));
#15679=DIRECTION('center_axis',(0.,0.,-1.));
#15680=DIRECTION('ref_axis',(0.,1.,0.));
#15681=DIRECTION('',(0.,1.,0.));
#15682=DIRECTION('',(1.,0.,0.));
#15683=DIRECTION('center_axis',(0.,1.,0.));
#15684=DIRECTION('ref_axis',(0.,0.,1.));
#15685=DIRECTION('',(0.,0.,1.));
#15686=DIRECTION('',(1.,0.,0.));
#15687=DIRECTION('center_axis',(0.,0.,-1.));
#15688=DIRECTION('ref_axis',(0.,1.,0.));
#15689=DIRECTION('',(0.,1.,0.));
#15690=DIRECTION('center_axis',(1.,0.,0.));
#15691=DIRECTION('ref_axis',(0.,0.,-1.));
#19419=CARTESIAN_POINT('',(0.,0.,0.));
#19420=CARTESIAN_POINT('Origin',(1.5,-1.9,1.7));
#19421=CARTESIAN_POINT('',(1.56403124237433,-1.7,1.7));
#19422=CARTESIAN_POINT('',(1.43596875762567,-1.7,1.7));
#19423=CARTESIAN_POINT('',(0.75,-1.7,1.7));
#19424=CARTESIAN_POINT('Origin',(1.5,-1.9,1.7));
#19425=CARTESIAN_POINT('Origin',(1.5,-1.9,1.7));
#19426=CARTESIAN_POINT('',(1.56403124237433,-1.7,1.75));
#19427=CARTESIAN_POINT('',(1.56403124237433,-1.7,1.7));
#19428=CARTESIAN_POINT('',(1.29,-1.9,1.75));
#19429=CARTESIAN_POINT('Origin',(1.5,-1.9,1.75));
#19430=CARTESIAN_POINT('',(1.29,-1.9,2.4));
#19431=CARTESIAN_POINT('',(1.29,-1.9,1.7));
#19432=CARTESIAN_POINT('Origin',(1.5,-1.9,2.4));
#19433=CARTESIAN_POINT('',(1.43596875762567,-1.7,1.75));
#19434=CARTESIAN_POINT('Origin',(1.5,-1.9,1.75));
#19435=CARTESIAN_POINT('',(1.43596875762567,-1.7,1.7));
#19436=CARTESIAN_POINT('Origin',(-1.5,1.9,1.7));
#19437=CARTESIAN_POINT('',(-1.56403124237433,1.7,1.7));
#19438=CARTESIAN_POINT('',(-1.43596875762567,1.7,1.7));
#19439=CARTESIAN_POINT('',(-0.75,1.7,1.7));
#19440=CARTESIAN_POINT('Origin',(-1.5,1.9,1.7));
#19441=CARTESIAN_POINT('Origin',(-1.5,1.9,1.7));
#19442=CARTESIAN_POINT('',(-1.56403124237433,1.7,1.75));
#19443=CARTESIAN_POINT('',(-1.56403124237433,1.7,1.7));
#19444=CARTESIAN_POINT('',(-1.71,1.9,1.75));
#19445=CARTESIAN_POINT('Origin',(-1.5,1.9,1.75));
#19446=CARTESIAN_POINT('',(-1.71,1.9,2.4));
#19447=CARTESIAN_POINT('',(-1.71,1.9,1.7));
#19448=CARTESIAN_POINT('Origin',(-1.5,1.9,2.4));
#19449=CARTESIAN_POINT('',(-1.43596875762567,1.7,1.75));
#19450=CARTESIAN_POINT('Origin',(-1.5,1.9,1.75));
#19451=CARTESIAN_POINT('',(-1.43596875762567,1.7,1.7));
#19452=CARTESIAN_POINT('Origin',(-1.5,-1.9,1.7));
#19453=CARTESIAN_POINT('',(-1.43596875762567,-1.7,1.7));
#19454=CARTESIAN_POINT('',(-1.56403124237433,-1.7,1.7));
#19455=CARTESIAN_POINT('',(-0.75,-1.7,1.7));
#19456=CARTESIAN_POINT('Origin',(-1.5,-1.9,1.7));
#19457=CARTESIAN_POINT('Origin',(-1.5,-1.9,1.7));
#19458=CARTESIAN_POINT('',(-1.43596875762567,-1.7,1.75));
#19459=CARTESIAN_POINT('',(-1.43596875762567,-1.7,1.7));
#19460=CARTESIAN_POINT('',(-1.71,-1.9,1.75));
#19461=CARTESIAN_POINT('Origin',(-1.5,-1.9,1.75));
#19462=CARTESIAN_POINT('',(-1.71,-1.9,2.4));
#19463=CARTESIAN_POINT('',(-1.71,-1.9,1.7));
#19464=CARTESIAN_POINT('Origin',(-1.5,-1.9,2.4));
#19465=CARTESIAN_POINT('',(-1.56403124237433,-1.7,1.75));
#19466=CARTESIAN_POINT('Origin',(-1.5,-1.9,1.75));
#19467=CARTESIAN_POINT('',(-1.56403124237433,-1.7,1.7));
#19468=CARTESIAN_POINT('Origin',(1.5,1.9,1.7));
#19469=CARTESIAN_POINT('',(1.43596875762567,1.7,1.7));
#19470=CARTESIAN_POINT('',(1.56403124237433,1.7,1.7));
#19471=CARTESIAN_POINT('',(0.75,1.7,1.7));
#19472=CARTESIAN_POINT('Origin',(1.5,1.9,1.7));
#19473=CARTESIAN_POINT('Origin',(1.5,1.9,1.7));
#19474=CARTESIAN_POINT('',(1.43596875762567,1.7,1.75));
#19475=CARTESIAN_POINT('',(1.43596875762567,1.7,1.7));
#19476=CARTESIAN_POINT('',(1.29,1.9,1.75));
#19477=CARTESIAN_POINT('Origin',(1.5,1.9,1.75));
#19478=CARTESIAN_POINT('',(1.29,1.9,2.4));
#19479=CARTESIAN_POINT('',(1.29,1.9,1.7));
#19480=CARTESIAN_POINT('Origin',(1.5,1.9,2.4));
#19481=CARTESIAN_POINT('',(1.56403124237433,1.7,1.75));
#19482=CARTESIAN_POINT('Origin',(1.5,1.9,1.75));
#19483=CARTESIAN_POINT('',(1.56403124237433,1.7,1.7));
#19484=CARTESIAN_POINT('Origin',(0.,-1.7,1.75));
#19485=CARTESIAN_POINT('',(0.,-1.7,1.75));
#19486=CARTESIAN_POINT('',(-1.97,-1.7,1.75));
#19487=CARTESIAN_POINT('',(0.,-1.7,1.75));
#19488=CARTESIAN_POINT('',(-1.97,-1.7,0.43));
#19489=CARTESIAN_POINT('',(-1.97,-1.7,1.75));
#19490=CARTESIAN_POINT('',(1.97,-1.7,0.43));
#19491=CARTESIAN_POINT('',(0.,-1.7,0.43));
#19492=CARTESIAN_POINT('',(1.97,-1.7,1.75));
#19493=CARTESIAN_POINT('',(1.97,-1.7,1.75));
#19494=CARTESIAN_POINT('',(0.,-1.7,1.75));
#19495=CARTESIAN_POINT('Origin',(0.,1.7,0.43));
#19496=CARTESIAN_POINT('',(0.,1.7,1.75));
#19497=CARTESIAN_POINT('',(1.97,1.7,1.75));
#19498=CARTESIAN_POINT('',(0.,1.7,1.75));
#19499=CARTESIAN_POINT('',(1.97,1.7,0.43));
#19500=CARTESIAN_POINT('',(1.97,1.7,0.43));
#19501=CARTESIAN_POINT('',(-1.97,1.7,0.43));
#19502=CARTESIAN_POINT('',(0.,1.7,0.43));
#19503=CARTESIAN_POINT('',(-1.97,1.7,1.75));
#19504=CARTESIAN_POINT('',(-1.97,1.7,0.43));
#19505=CARTESIAN_POINT('',(0.,1.7,1.75));
#19506=CARTESIAN_POINT('Origin',(-1.97,0.,1.415));
#19507=CARTESIAN_POINT('',(-1.97,-2.35,1.75));
#19508=CARTESIAN_POINT('',(-1.97,-2.35,1.75));
#19509=CARTESIAN_POINT('',(-1.97,-2.35,2.4));
#19510=CARTESIAN_POINT('',(-1.97,-2.35,2.4));
#19511=CARTESIAN_POINT('',(-1.97,2.35,2.4));
#19512=CARTESIAN_POINT('',(-1.97,2.35,2.4));
#19513=CARTESIAN_POINT('',(-1.97,2.35,1.75));
#19514=CARTESIAN_POINT('',(-1.97,2.35,1.75));
#19515=CARTESIAN_POINT('',(-1.97,1.7,1.75));
#19516=CARTESIAN_POINT('',(-1.97,0.78,0.43));
#19517=CARTESIAN_POINT('',(-1.97,0.78,0.43));
#19518=CARTESIAN_POINT('',(-1.97,0.78,1.55));
#19519=CARTESIAN_POINT('',(-1.97,0.78,1.55));
#19520=CARTESIAN_POINT('',(-1.97,-0.78,1.55));
#19521=CARTESIAN_POINT('',(-1.97,-0.78,1.55));
#19522=CARTESIAN_POINT('',(-1.97,-0.78,0.43));
#19523=CARTESIAN_POINT('',(-1.97,-0.78,0.43));
#19524=CARTESIAN_POINT('',(-1.97,-1.7,0.43));
#19525=CARTESIAN_POINT('Origin',(0.,-2.35,1.75));
#19526=CARTESIAN_POINT('',(1.97,-2.35,1.75));
#19527=CARTESIAN_POINT('',(1.97,-2.35,1.75));
#19528=CARTESIAN_POINT('',(0.,-2.35,1.75));
#19529=CARTESIAN_POINT('Origin',(0.,-2.35,2.4));
#19530=CARTESIAN_POINT('',(1.97,-2.35,2.4));
#19531=CARTESIAN_POINT('',(1.97,-2.35,2.4));
#19532=CARTESIAN_POINT('',(0.,-2.35,2.4));
#19533=CARTESIAN_POINT('Origin',(0.,2.35,2.4));
#19534=CARTESIAN_POINT('',(1.97,2.35,2.4));
#19535=CARTESIAN_POINT('',(1.97,2.35,2.4));
#19536=CARTESIAN_POINT('',(0.,2.35,2.4));
#19537=CARTESIAN_POINT('Origin',(0.,2.35,1.75));
#19538=CARTESIAN_POINT('',(1.97,2.35,1.75));
#19539=CARTESIAN_POINT('',(1.97,2.35,1.75));
#19540=CARTESIAN_POINT('',(0.,2.35,1.75));
#19541=CARTESIAN_POINT('Origin',(0.,1.7,1.75));
#19542=CARTESIAN_POINT('',(1.97,1.7,1.75));
#19543=CARTESIAN_POINT('Origin',(0.,0.78,0.43));
#19544=CARTESIAN_POINT('',(1.97,0.78,0.43));
#19545=CARTESIAN_POINT('',(1.97,0.78,0.43));
#19546=CARTESIAN_POINT('',(0.,0.78,0.43));
#19547=CARTESIAN_POINT('Origin',(0.,0.78,1.55));
#19548=CARTESIAN_POINT('',(1.97,0.78,1.55));
#19549=CARTESIAN_POINT('',(1.97,0.78,1.55));
#19550=CARTESIAN_POINT('',(0.,0.78,1.55));
#19551=CARTESIAN_POINT('Origin',(0.,-0.78,1.55));
#19552=CARTESIAN_POINT('',(1.97,-0.78,1.55));
#19553=CARTESIAN_POINT('',(1.97,-0.78,1.55));
#19554=CARTESIAN_POINT('',(0.,-0.78,1.55));
#19555=CARTESIAN_POINT('Origin',(0.,-0.78,0.43));
#19556=CARTESIAN_POINT('',(1.97,-0.78,0.43));
#19557=CARTESIAN_POINT('',(1.97,-0.78,0.43));
#19558=CARTESIAN_POINT('',(0.,-0.78,0.43));
#19559=CARTESIAN_POINT('Origin',(0.,-1.7,0.43));
#19560=CARTESIAN_POINT('',(1.97,-1.7,0.43));
#19561=CARTESIAN_POINT('Origin',(1.97,0.,1.415));
#20035=UNCERTAINTY_MEASURE_WITH_UNIT(LENGTH_MEASURE(0.001),#20097,
'DISTANCE_ACCURACY_VALUE',
'Maximum model space distance between geometric entities at asserted c
onnectivities');
#20042=UNCERTAINTY_MEASURE_WITH_UNIT(LENGTH_MEASURE(0.001),#20097,
'DISTANCE_ACCURACY_VALUE',
'Maximum model space distance between geometric entities at asserted c
onnectivities');
#20089=(
GEOMETRIC_REPRESENTATION_CONTEXT(3)
GLOBAL_UNCERTAINTY_ASSIGNED_CONTEXT((#20035))
GLOBAL_UNIT_ASSIGNED_CONTEXT((#20097,#20099,#20100))
REPRESENTATION_CONTEXT('','3D')
);
#20096=(
GEOMETRIC_REPRESENTATION_CONTEXT(3)
GLOBAL_UNCERTAINTY_ASSIGNED_CONTEXT((#20042))
GLOBAL_UNIT_ASSIGNED_CONTEXT((#20097,#20099,#20100))
REPRESENTATION_CONTEXT('','3D')
);
#20097=(
LENGTH_UNIT()
NAMED_UNIT(*)
SI_UNIT(.CENTI.,.METRE.)
);
#20099=(
NAMED_UNIT(*)
PLANE_ANGLE_UNIT()
SI_UNIT($,.RADIAN.)
);
#20100=(
NAMED_UNIT(*)
SI_UNIT($,.STERADIAN.)
SOLID_ANGLE_UNIT()
);
#20147=SHAPE_DEFINITION_REPRESENTATION(#20205,#20358);
#20205=PRODUCT_DEFINITION_SHAPE('',$,#20412);
#20358=SHAPE_REPRESENTATION('',(#12537),#20089);
#20365=PRODUCT_DEFINITION_CONTEXT('part definition',#20526,'design');
#20412=PRODUCT_DEFINITION('Block','Block',#20465,#20365);
#20465=PRODUCT_DEFINITION_FORMATION('',$,#20574);
#20526=APPLICATION_CONTEXT(
'Core Data for Automotive Mechanical Design Process');
#20527=PRODUCT_CONTEXT('part definition',#20526,'mechanical');
#20574=PRODUCT('Block','Block','Block',(#20527));
#20623=COLOUR_RGB('Dark Blue',0.08,0.2,0.34);
#20624=FILL_AREA_STYLE_COLOUR('',#20623);
#20625=FILL_AREA_STYLE('',(#20624));
#20626=SURFACE_STYLE_FILL_AREA(#20625);
#20627=SURFACE_SIDE_STYLE('',(#20626));
#20628=SURFACE_STYLE_USAGE(.BOTH.,#20627);
#20629=PRESENTATION_STYLE_ASSIGNMENT((#20628));
ENDSEC;
END-ISO-10303-21;
